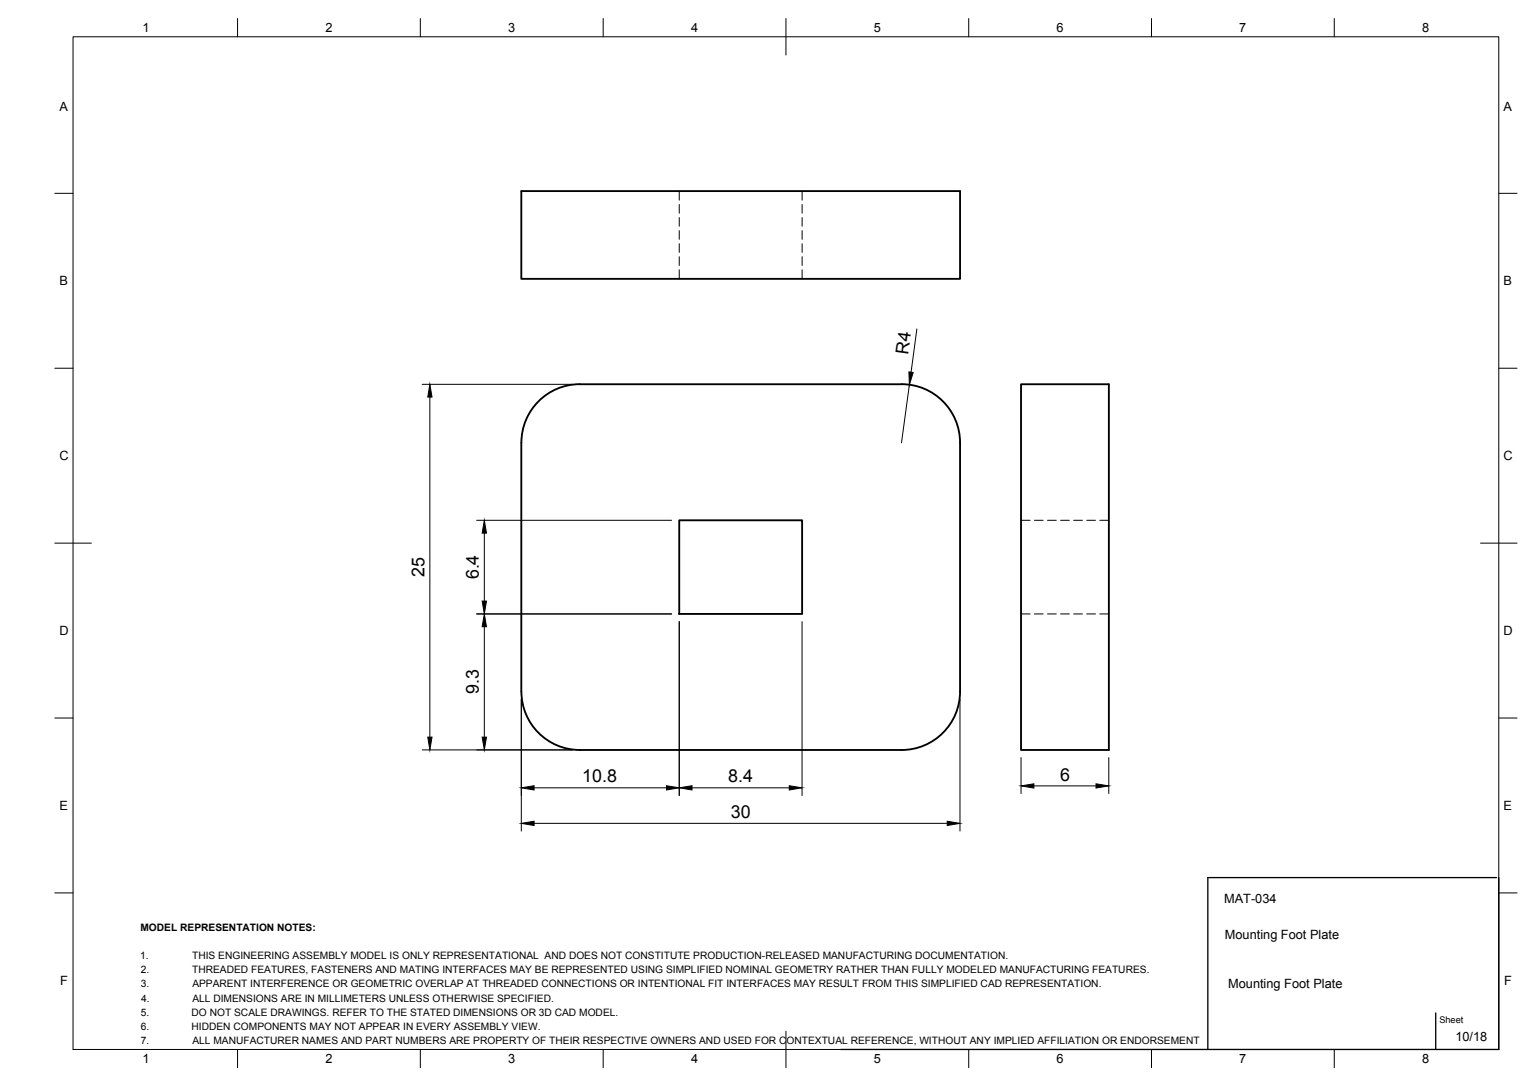
ISO-10303-21;
HEADER;
/* Generated by software containing ST-Developer
 * from STEP Tools, Inc. (www.steptools.com) 
 */

FILE_DESCRIPTION(
/* description */ ('STEP AP214'),
/* implementation_level */ '2;1');

FILE_NAME(
/* name */ 'Mounting Foot Plate.step',
/* time_stamp */ '2026-11-14T09:24:36-08:00',
/* author */ (''),
/* organization */ (''),
/* preprocessor_version */ 'ST-DEVELOPER v20.2',
/* originating_system */ 'Autodesk Translation Framework v15.17.0.0',
/* authorisation */ '');

FILE_SCHEMA (('AUTOMOTIVE_DESIGN { 1 0 10303 214 3 1 1 }'));
ENDSEC;

DATA;
#10=MECHANICAL_DESIGN_GEOMETRIC_PRESENTATION_REPRESENTATION('',(#216),#18867);
#184=SHAPE_REPRESENTATION_RELATIONSHIP('SRR','None',#18948,#200);
#200=ADVANCED_BREP_SHAPE_REPRESENTATION('',(#240),#18864);
#216=STYLED_ITEM('',(#19024),#240);
#240=MANIFOLD_SOLID_BREP('Body1',#10971);
#365=FACE_BOUND('',#1958,.T.);
#366=FACE_BOUND('',#1960,.T.);
#701=PLANE('',#12113);
#702=PLANE('',#12118);
#703=PLANE('',#12123);
#704=PLANE('',#12124);
#705=PLANE('',#12125);
#706=PLANE('',#12126);
#707=PLANE('',#12127);
#708=PLANE('',#12128);
#709=PLANE('',#12129);
#710=PLANE('',#12130);
#1247=FACE_OUTER_BOUND('',#1957,.T.);
#1248=FACE_OUTER_BOUND('',#1959,.T.);
#1249=FACE_OUTER_BOUND('',#1961,.T.);
#1250=FACE_OUTER_BOUND('',#1962,.T.);
#1251=FACE_OUTER_BOUND('',#1963,.T.);
#1252=FACE_OUTER_BOUND('',#1964,.T.);
#1253=FACE_OUTER_BOUND('',#1965,.T.);
#1254=FACE_OUTER_BOUND('',#1966,.T.);
#1255=FACE_OUTER_BOUND('',#1967,.T.);
#1256=FACE_OUTER_BOUND('',#1968,.T.);
#1257=FACE_OUTER_BOUND('',#1969,.T.);
#1258=FACE_OUTER_BOUND('',#1970,.T.);
#1259=FACE_OUTER_BOUND('',#1971,.T.);
#1260=FACE_OUTER_BOUND('',#1972,.T.);
#1957=EDGE_LOOP('',(#9864,#9865,#9866,#9867,#9868,#9869,#9870,#9871));
#1958=EDGE_LOOP('',(#9872,#9873,#9874,#9875));
#1959=EDGE_LOOP('',(#9876,#9877,#9878,#9879,#9880,#9881,#9882,#9883));
#1960=EDGE_LOOP('',(#9884,#9885,#9886,#9887));
#1961=EDGE_LOOP('',(#9888,#9889,#9890,#9891));
#1962=EDGE_LOOP('',(#9892,#9893,#9894,#9895));
#1963=EDGE_LOOP('',(#9896,#9897,#9898,#9899));
#1964=EDGE_LOOP('',(#9900,#9901,#9902,#9903));
#1965=EDGE_LOOP('',(#9904,#9905,#9906,#9907));
#1966=EDGE_LOOP('',(#9908,#9909,#9910,#9911));
#1967=EDGE_LOOP('',(#9912,#9913,#9914,#9915));
#1968=EDGE_LOOP('',(#9916,#9917,#9918,#9919));
#1969=EDGE_LOOP('',(#9920,#9921,#9922,#9923));
#1970=EDGE_LOOP('',(#9924,#9925,#9926,#9927));
#1971=EDGE_LOOP('',(#9928,#9929,#9930,#9931));
#1972=EDGE_LOOP('',(#9932,#9933,#9934,#9935));
#3004=LINE('',#18489,#4018);
#3005=LINE('',#18493,#4019);
#3006=LINE('',#18497,#4020);
#3007=LINE('',#18501,#4021);
#3008=LINE('',#18505,#4022);
#3009=LINE('',#18507,#4023);
#3010=LINE('',#18509,#4024);
#3011=LINE('',#18510,#4025);
#3012=LINE('',#18514,#4026);
#3013=LINE('',#18518,#4027);
#3014=LINE('',#18522,#4028);
#3015=LINE('',#18526,#4029);
#3016=LINE('',#18530,#4030);
#3017=LINE('',#18532,#4031);
#3018=LINE('',#18534,#4032);
#3019=LINE('',#18535,#4033);
#3020=LINE('',#18537,#4034);
#3021=LINE('',#18538,#4035);
#3022=LINE('',#18540,#4036);
#3023=LINE('',#18541,#4037);
#3024=LINE('',#18543,#4038);
#3025=LINE('',#18544,#4039);
#3026=LINE('',#18546,#4040);
#3027=LINE('',#18547,#4041);
#3028=LINE('',#18549,#4042);
#3029=LINE('',#18550,#4043);
#3030=LINE('',#18552,#4044);
#3031=LINE('',#18554,#4045);
#4018=VECTOR('',#15170,1000.);
#4019=VECTOR('',#15173,1000.);
#4020=VECTOR('',#15176,1000.);
#4021=VECTOR('',#15179,1000.);
#4022=VECTOR('',#15182,1000.);
#4023=VECTOR('',#15183,1000.);
#4024=VECTOR('',#15184,1000.);
#4025=VECTOR('',#15185,1000.);
#4026=VECTOR('',#15188,1000.);
#4027=VECTOR('',#15191,1000.);
#4028=VECTOR('',#15194,1000.);
#4029=VECTOR('',#15197,1000.);
#4030=VECTOR('',#15200,1000.);
#4031=VECTOR('',#15201,1000.);
#4032=VECTOR('',#15202,1000.);
#4033=VECTOR('',#15203,1000.);
#4034=VECTOR('',#15206,1000.);
#4035=VECTOR('',#15207,1000.);
#4036=VECTOR('',#15210,1000.);
#4037=VECTOR('',#15211,1000.);
#4038=VECTOR('',#15214,1000.);
#4039=VECTOR('',#15215,1000.);
#4040=VECTOR('',#15218,1000.);
#4041=VECTOR('',#15219,1000.);
#4042=VECTOR('',#15222,1000.);
#4043=VECTOR('',#15223,1000.);
#4044=VECTOR('',#15226,1000.);
#4045=VECTOR('',#15229,1000.);
#4488=CIRCLE('',#12114,4.);
#4489=CIRCLE('',#12115,4.);
#4490=CIRCLE('',#12116,4.);
#4491=CIRCLE('',#12117,4.);
#4492=CIRCLE('',#12119,4.);
#4493=CIRCLE('',#12120,4.);
#4494=CIRCLE('',#12121,4.);
#4495=CIRCLE('',#12122,4.);
#5488=VERTEX_POINT('',#18487);
#5489=VERTEX_POINT('',#18488);
#5490=VERTEX_POINT('',#18490);
#5491=VERTEX_POINT('',#18492);
#5492=VERTEX_POINT('',#18494);
#5493=VERTEX_POINT('',#18496);
#5494=VERTEX_POINT('',#18498);
#5495=VERTEX_POINT('',#18500);
#5496=VERTEX_POINT('',#18503);
#5497=VERTEX_POINT('',#18504);
#5498=VERTEX_POINT('',#18506);
#5499=VERTEX_POINT('',#18508);
#5500=VERTEX_POINT('',#18512);
#5501=VERTEX_POINT('',#18513);
#5502=VERTEX_POINT('',#18515);
#5503=VERTEX_POINT('',#18517);
#5504=VERTEX_POINT('',#18519);
#5505=VERTEX_POINT('',#18521);
#5506=VERTEX_POINT('',#18523);
#5507=VERTEX_POINT('',#18525);
#5508=VERTEX_POINT('',#18528);
#5509=VERTEX_POINT('',#18529);
#5510=VERTEX_POINT('',#18531);
#5511=VERTEX_POINT('',#18533);
#6965=EDGE_CURVE('',#5488,#5489,#3004,.T.);
#6966=EDGE_CURVE('',#5489,#5490,#4488,.T.);
#6967=EDGE_CURVE('',#5490,#5491,#3005,.T.);
#6968=EDGE_CURVE('',#5491,#5492,#4489,.T.);
#6969=EDGE_CURVE('',#5492,#5493,#3006,.T.);
#6970=EDGE_CURVE('',#5493,#5494,#4490,.T.);
#6971=EDGE_CURVE('',#5494,#5495,#3007,.T.);
#6972=EDGE_CURVE('',#5495,#5488,#4491,.T.);
#6973=EDGE_CURVE('',#5496,#5497,#3008,.T.);
#6974=EDGE_CURVE('',#5498,#5496,#3009,.T.);
#6975=EDGE_CURVE('',#5499,#5498,#3010,.T.);
#6976=EDGE_CURVE('',#5497,#5499,#3011,.T.);
#6977=EDGE_CURVE('',#5500,#5501,#3012,.T.);
#6978=EDGE_CURVE('',#5500,#5502,#4492,.T.);
#6979=EDGE_CURVE('',#5503,#5502,#3013,.T.);
#6980=EDGE_CURVE('',#5503,#5504,#4493,.T.);
#6981=EDGE_CURVE('',#5505,#5504,#3014,.T.);
#6982=EDGE_CURVE('',#5505,#5506,#4494,.T.);
#6983=EDGE_CURVE('',#5507,#5506,#3015,.T.);
#6984=EDGE_CURVE('',#5507,#5501,#4495,.T.);
#6985=EDGE_CURVE('',#5508,#5509,#3016,.T.);
#6986=EDGE_CURVE('',#5509,#5510,#3017,.T.);
#6987=EDGE_CURVE('',#5510,#5511,#3018,.T.);
#6988=EDGE_CURVE('',#5511,#5508,#3019,.T.);
#6989=EDGE_CURVE('',#5490,#5500,#3020,.T.);
#6990=EDGE_CURVE('',#5501,#5491,#3021,.T.);
#6991=EDGE_CURVE('',#5492,#5507,#3022,.T.);
#6992=EDGE_CURVE('',#5506,#5493,#3023,.T.);
#6993=EDGE_CURVE('',#5504,#5495,#3024,.T.);
#6994=EDGE_CURVE('',#5494,#5505,#3025,.T.);
#6995=EDGE_CURVE('',#5502,#5489,#3026,.T.);
#6996=EDGE_CURVE('',#5488,#5503,#3027,.T.);
#6997=EDGE_CURVE('',#5498,#5508,#3028,.T.);
#6998=EDGE_CURVE('',#5496,#5509,#3029,.T.);
#6999=EDGE_CURVE('',#5497,#5510,#3030,.T.);
#7000=EDGE_CURVE('',#5499,#5511,#3031,.T.);
#9864=ORIENTED_EDGE('',*,*,#6965,.T.);
#9865=ORIENTED_EDGE('',*,*,#6966,.T.);
#9866=ORIENTED_EDGE('',*,*,#6967,.T.);
#9867=ORIENTED_EDGE('',*,*,#6968,.T.);
#9868=ORIENTED_EDGE('',*,*,#6969,.T.);
#9869=ORIENTED_EDGE('',*,*,#6970,.T.);
#9870=ORIENTED_EDGE('',*,*,#6971,.T.);
#9871=ORIENTED_EDGE('',*,*,#6972,.T.);
#9872=ORIENTED_EDGE('',*,*,#6973,.F.);
#9873=ORIENTED_EDGE('',*,*,#6974,.F.);
#9874=ORIENTED_EDGE('',*,*,#6975,.F.);
#9875=ORIENTED_EDGE('',*,*,#6976,.F.);
#9876=ORIENTED_EDGE('',*,*,#6977,.F.);
#9877=ORIENTED_EDGE('',*,*,#6978,.T.);
#9878=ORIENTED_EDGE('',*,*,#6979,.F.);
#9879=ORIENTED_EDGE('',*,*,#6980,.T.);
#9880=ORIENTED_EDGE('',*,*,#6981,.F.);
#9881=ORIENTED_EDGE('',*,*,#6982,.T.);
#9882=ORIENTED_EDGE('',*,*,#6983,.F.);
#9883=ORIENTED_EDGE('',*,*,#6984,.T.);
#9884=ORIENTED_EDGE('',*,*,#6985,.T.);
#9885=ORIENTED_EDGE('',*,*,#6986,.T.);
#9886=ORIENTED_EDGE('',*,*,#6987,.T.);
#9887=ORIENTED_EDGE('',*,*,#6988,.T.);
#9888=ORIENTED_EDGE('',*,*,#6967,.F.);
#9889=ORIENTED_EDGE('',*,*,#6989,.T.);
#9890=ORIENTED_EDGE('',*,*,#6977,.T.);
#9891=ORIENTED_EDGE('',*,*,#6990,.T.);
#9892=ORIENTED_EDGE('',*,*,#6969,.F.);
#9893=ORIENTED_EDGE('',*,*,#6991,.T.);
#9894=ORIENTED_EDGE('',*,*,#6983,.T.);
#9895=ORIENTED_EDGE('',*,*,#6992,.T.);
#9896=ORIENTED_EDGE('',*,*,#6981,.T.);
#9897=ORIENTED_EDGE('',*,*,#6993,.T.);
#9898=ORIENTED_EDGE('',*,*,#6971,.F.);
#9899=ORIENTED_EDGE('',*,*,#6994,.T.);
#9900=ORIENTED_EDGE('',*,*,#6979,.T.);
#9901=ORIENTED_EDGE('',*,*,#6995,.T.);
#9902=ORIENTED_EDGE('',*,*,#6965,.F.);
#9903=ORIENTED_EDGE('',*,*,#6996,.T.);
#9904=ORIENTED_EDGE('',*,*,#6985,.F.);
#9905=ORIENTED_EDGE('',*,*,#6997,.F.);
#9906=ORIENTED_EDGE('',*,*,#6974,.T.);
#9907=ORIENTED_EDGE('',*,*,#6998,.T.);
#9908=ORIENTED_EDGE('',*,*,#6986,.F.);
#9909=ORIENTED_EDGE('',*,*,#6998,.F.);
#9910=ORIENTED_EDGE('',*,*,#6973,.T.);
#9911=ORIENTED_EDGE('',*,*,#6999,.T.);
#9912=ORIENTED_EDGE('',*,*,#6987,.F.);
#9913=ORIENTED_EDGE('',*,*,#6999,.F.);
#9914=ORIENTED_EDGE('',*,*,#6976,.T.);
#9915=ORIENTED_EDGE('',*,*,#7000,.T.);
#9916=ORIENTED_EDGE('',*,*,#6988,.F.);
#9917=ORIENTED_EDGE('',*,*,#7000,.F.);
#9918=ORIENTED_EDGE('',*,*,#6975,.T.);
#9919=ORIENTED_EDGE('',*,*,#6997,.T.);
#9920=ORIENTED_EDGE('',*,*,#6966,.F.);
#9921=ORIENTED_EDGE('',*,*,#6995,.F.);
#9922=ORIENTED_EDGE('',*,*,#6978,.F.);
#9923=ORIENTED_EDGE('',*,*,#6989,.F.);
#9924=ORIENTED_EDGE('',*,*,#6972,.F.);
#9925=ORIENTED_EDGE('',*,*,#6993,.F.);
#9926=ORIENTED_EDGE('',*,*,#6980,.F.);
#9927=ORIENTED_EDGE('',*,*,#6996,.F.);
#9928=ORIENTED_EDGE('',*,*,#6968,.F.);
#9929=ORIENTED_EDGE('',*,*,#6990,.F.);
#9930=ORIENTED_EDGE('',*,*,#6984,.F.);
#9931=ORIENTED_EDGE('',*,*,#6991,.F.);
#9932=ORIENTED_EDGE('',*,*,#6970,.F.);
#9933=ORIENTED_EDGE('',*,*,#6992,.F.);
#9934=ORIENTED_EDGE('',*,*,#6982,.F.);
#9935=ORIENTED_EDGE('',*,*,#6994,.F.);
#10341=CYLINDRICAL_SURFACE('',#12131,4.);
#10342=CYLINDRICAL_SURFACE('',#12132,4.);
#10343=CYLINDRICAL_SURFACE('',#12133,4.);
#10344=CYLINDRICAL_SURFACE('',#12134,4.);
#10884=ADVANCED_FACE('',(#1247,#365),#701,.T.);
#10885=ADVANCED_FACE('',(#1248,#366),#702,.F.);
#10886=ADVANCED_FACE('',(#1249),#703,.F.);
#10887=ADVANCED_FACE('',(#1250),#704,.F.);
#10888=ADVANCED_FACE('',(#1251),#705,.F.);
#10889=ADVANCED_FACE('',(#1252),#706,.F.);
#10890=ADVANCED_FACE('',(#1253),#707,.T.);
#10891=ADVANCED_FACE('',(#1254),#708,.T.);
#10892=ADVANCED_FACE('',(#1255),#709,.T.);
#10893=ADVANCED_FACE('',(#1256),#710,.T.);
#10894=ADVANCED_FACE('',(#1257),#10341,.T.);
#10895=ADVANCED_FACE('',(#1258),#10342,.T.);
#10896=ADVANCED_FACE('',(#1259),#10343,.T.);
#10897=ADVANCED_FACE('',(#1260),#10344,.T.);
#10971=CLOSED_SHELL('',(#10884,#10885,#10886,#10887,#10888,#10889,#10890,
#10891,#10892,#10893,#10894,#10895,#10896,#10897));
#12112=AXIS2_PLACEMENT_3D('',#18485,#15166,#15167);
#12113=AXIS2_PLACEMENT_3D('',#18486,#15168,#15169);
#12114=AXIS2_PLACEMENT_3D('',#18491,#15171,#15172);
#12115=AXIS2_PLACEMENT_3D('',#18495,#15174,#15175);
#12116=AXIS2_PLACEMENT_3D('',#18499,#15177,#15178);
#12117=AXIS2_PLACEMENT_3D('',#18502,#15180,#15181);
#12118=AXIS2_PLACEMENT_3D('',#18511,#15186,#15187);
#12119=AXIS2_PLACEMENT_3D('',#18516,#15189,#15190);
#12120=AXIS2_PLACEMENT_3D('',#18520,#15192,#15193);
#12121=AXIS2_PLACEMENT_3D('',#18524,#15195,#15196);
#12122=AXIS2_PLACEMENT_3D('',#18527,#15198,#15199);
#12123=AXIS2_PLACEMENT_3D('',#18536,#15204,#15205);
#12124=AXIS2_PLACEMENT_3D('',#18539,#15208,#15209);
#12125=AXIS2_PLACEMENT_3D('',#18542,#15212,#15213);
#12126=AXIS2_PLACEMENT_3D('',#18545,#15216,#15217);
#12127=AXIS2_PLACEMENT_3D('',#18548,#15220,#15221);
#12128=AXIS2_PLACEMENT_3D('',#18551,#15224,#15225);
#12129=AXIS2_PLACEMENT_3D('',#18553,#15227,#15228);
#12130=AXIS2_PLACEMENT_3D('',#18555,#15230,#15231);
#12131=AXIS2_PLACEMENT_3D('',#18556,#15232,#15233);
#12132=AXIS2_PLACEMENT_3D('',#18557,#15234,#15235);
#12133=AXIS2_PLACEMENT_3D('',#18558,#15236,#15237);
#12134=AXIS2_PLACEMENT_3D('',#18559,#15238,#15239);
#15166=DIRECTION('axis',(0.,0.,1.));
#15167=DIRECTION('refdir',(1.,0.,0.));
#15168=DIRECTION('center_axis',(0.,1.,0.));
#15169=DIRECTION('ref_axis',(0.,0.,1.));
#15170=DIRECTION('',(-1.,0.,1.15648231731787E-16));
#15171=DIRECTION('center_axis',(0.,1.,0.));
#15172=DIRECTION('ref_axis',(0.,0.,1.));
#15173=DIRECTION('',(0.,0.,1.));
#15174=DIRECTION('center_axis',(0.,1.,0.));
#15175=DIRECTION('ref_axis',(0.,0.,1.));
#15176=DIRECTION('',(1.,0.,-1.15648231731787E-16));
#15177=DIRECTION('center_axis',(0.,1.,0.));
#15178=DIRECTION('ref_axis',(0.,0.,1.));
#15179=DIRECTION('',(0.,0.,-1.));
#15180=DIRECTION('center_axis',(0.,1.,0.));
#15181=DIRECTION('ref_axis',(0.,0.,1.));
#15182=DIRECTION('',(1.,0.,-1.03257349760524E-16));
#15183=DIRECTION('',(0.,0.,1.));
#15184=DIRECTION('',(-1.,0.,1.03257349760524E-16));
#15185=DIRECTION('',(0.,0.,-1.));
#15186=DIRECTION('center_axis',(0.,1.,0.));
#15187=DIRECTION('ref_axis',(0.,0.,1.));
#15188=DIRECTION('',(0.,0.,1.));
#15189=DIRECTION('center_axis',(0.,-1.,0.));
#15190=DIRECTION('ref_axis',(0.,0.,1.));
#15191=DIRECTION('',(-1.,0.,1.15648231731787E-16));
#15192=DIRECTION('center_axis',(0.,-1.,0.));
#15193=DIRECTION('ref_axis',(0.,0.,1.));
#15194=DIRECTION('',(0.,0.,-1.));
#15195=DIRECTION('center_axis',(0.,-1.,0.));
#15196=DIRECTION('ref_axis',(0.,0.,1.));
#15197=DIRECTION('',(1.,0.,-1.15648231731787E-16));
#15198=DIRECTION('center_axis',(0.,-1.,0.));
#15199=DIRECTION('ref_axis',(0.,0.,1.));
#15200=DIRECTION('',(0.,0.,1.));
#15201=DIRECTION('',(1.,0.,-1.03257349760524E-16));
#15202=DIRECTION('',(0.,0.,-1.));
#15203=DIRECTION('',(-1.,0.,1.03257349760524E-16));
#15204=DIRECTION('center_axis',(1.,0.,0.));
#15205=DIRECTION('ref_axis',(0.,0.,-1.));
#15206=DIRECTION('',(0.,-1.,0.));
#15207=DIRECTION('',(0.,1.,0.));
#15208=DIRECTION('center_axis',(-1.15648231731787E-16,0.,-1.));
#15209=DIRECTION('ref_axis',(-1.,0.,1.15648231731787E-16));
#15210=DIRECTION('',(0.,-1.,0.));
#15211=DIRECTION('',(0.,1.,0.));
#15212=DIRECTION('center_axis',(-1.,0.,0.));
#15213=DIRECTION('ref_axis',(0.,0.,1.));
#15214=DIRECTION('',(0.,1.,0.));
#15215=DIRECTION('',(0.,-1.,0.));
#15216=DIRECTION('center_axis',(1.15648231731787E-16,0.,1.));
#15217=DIRECTION('ref_axis',(1.,0.,-1.15648231731787E-16));
#15218=DIRECTION('',(0.,1.,0.));
#15219=DIRECTION('',(0.,-1.,0.));
#15220=DIRECTION('center_axis',(1.,0.,0.));
#15221=DIRECTION('ref_axis',(0.,0.,-1.));
#15222=DIRECTION('',(0.,-1.,0.));
#15223=DIRECTION('',(0.,-1.,0.));
#15224=DIRECTION('center_axis',(-1.03257349760524E-16,0.,-1.));
#15225=DIRECTION('ref_axis',(-1.,0.,1.03257349760524E-16));
#15226=DIRECTION('',(0.,-1.,0.));
#15227=DIRECTION('center_axis',(-1.,0.,0.));
#15228=DIRECTION('ref_axis',(0.,0.,1.));
#15229=DIRECTION('',(0.,-1.,0.));
#15230=DIRECTION('center_axis',(1.03257349760524E-16,0.,1.));
#15231=DIRECTION('ref_axis',(1.,0.,-1.03257349760524E-16));
#15232=DIRECTION('center_axis',(0.,-1.,0.));
#15233=DIRECTION('ref_axis',(0.,0.,-1.));
#15234=DIRECTION('center_axis',(0.,-1.,0.));
#15235=DIRECTION('ref_axis',(0.,0.,-1.));
#15236=DIRECTION('center_axis',(0.,-1.,0.));
#15237=DIRECTION('ref_axis',(0.,0.,-1.));
#15238=DIRECTION('center_axis',(0.,-1.,0.));
#15239=DIRECTION('ref_axis',(0.,0.,-1.));
#18485=CARTESIAN_POINT('',(0.,0.,0.));
#18486=CARTESIAN_POINT('Origin',(0.,6.,0.));
#18487=CARTESIAN_POINT('',(11.,6.,-12.5));
#18488=CARTESIAN_POINT('',(-11.,6.,-12.5));
#18489=CARTESIAN_POINT('',(15.,6.,-12.5));
#18490=CARTESIAN_POINT('',(-15.,6.,-8.49999999999999));
#18491=CARTESIAN_POINT('Origin',(-11.,6.,-8.49999999999999));
#18492=CARTESIAN_POINT('',(-15.,6.,8.50000000000001));
#18493=CARTESIAN_POINT('',(-15.,6.,12.5));
#18494=CARTESIAN_POINT('',(-11.,6.,12.5));
#18495=CARTESIAN_POINT('Origin',(-11.,6.,8.50000000000001));
#18496=CARTESIAN_POINT('',(11.,6.,12.5));
#18497=CARTESIAN_POINT('',(15.,6.,12.5));
#18498=CARTESIAN_POINT('',(15.,6.,8.5));
#18499=CARTESIAN_POINT('Origin',(11.,6.,8.5));
#18500=CARTESIAN_POINT('',(15.,6.,-8.5));
#18501=CARTESIAN_POINT('',(15.,6.,12.5));
#18502=CARTESIAN_POINT('Origin',(11.,6.,-8.5));
#18503=CARTESIAN_POINT('',(-4.2,6.,3.2));
#18504=CARTESIAN_POINT('',(4.2,6.,3.2));
#18505=CARTESIAN_POINT('',(4.2,6.,3.2));
#18506=CARTESIAN_POINT('',(-4.2,6.,-3.2));
#18507=CARTESIAN_POINT('',(-4.2,6.,3.2));
#18508=CARTESIAN_POINT('',(4.2,6.,-3.2));
#18509=CARTESIAN_POINT('',(4.2,6.,-3.2));
#18510=CARTESIAN_POINT('',(4.2,6.,3.2));
#18511=CARTESIAN_POINT('Origin',(0.,0.,0.));
#18512=CARTESIAN_POINT('',(-15.,0.,-8.49999999999999));
#18513=CARTESIAN_POINT('',(-15.,0.,8.50000000000001));
#18514=CARTESIAN_POINT('',(-15.,0.,12.5));
#18515=CARTESIAN_POINT('',(-11.,0.,-12.5));
#18516=CARTESIAN_POINT('Origin',(-11.,0.,-8.49999999999999));
#18517=CARTESIAN_POINT('',(11.,0.,-12.5));
#18518=CARTESIAN_POINT('',(15.,0.,-12.5));
#18519=CARTESIAN_POINT('',(15.,0.,-8.5));
#18520=CARTESIAN_POINT('Origin',(11.,0.,-8.5));
#18521=CARTESIAN_POINT('',(15.,0.,8.5));
#18522=CARTESIAN_POINT('',(15.,0.,12.5));
#18523=CARTESIAN_POINT('',(11.,0.,12.5));
#18524=CARTESIAN_POINT('Origin',(11.,0.,8.5));
#18525=CARTESIAN_POINT('',(-11.,0.,12.5));
#18526=CARTESIAN_POINT('',(15.,0.,12.5));
#18527=CARTESIAN_POINT('Origin',(-11.,0.,8.50000000000001));
#18528=CARTESIAN_POINT('',(-4.2,0.,-3.2));
#18529=CARTESIAN_POINT('',(-4.2,0.,3.2));
#18530=CARTESIAN_POINT('',(-4.2,0.,3.2));
#18531=CARTESIAN_POINT('',(4.2,0.,3.2));
#18532=CARTESIAN_POINT('',(4.2,0.,3.2));
#18533=CARTESIAN_POINT('',(4.2,0.,-3.2));
#18534=CARTESIAN_POINT('',(4.2,0.,3.2));
#18535=CARTESIAN_POINT('',(4.2,0.,-3.2));
#18536=CARTESIAN_POINT('Origin',(-15.,6.,12.5));
#18537=CARTESIAN_POINT('',(-15.,6.,-8.49999999999999));
#18538=CARTESIAN_POINT('',(-15.,6.,8.50000000000001));
#18539=CARTESIAN_POINT('Origin',(15.,6.,12.5));
#18540=CARTESIAN_POINT('',(-11.,6.,12.5));
#18541=CARTESIAN_POINT('',(11.,6.,12.5));
#18542=CARTESIAN_POINT('Origin',(15.,6.,12.5));
#18543=CARTESIAN_POINT('',(15.,6.,-8.5));
#18544=CARTESIAN_POINT('',(15.,6.,8.5));
#18545=CARTESIAN_POINT('Origin',(15.,6.,-12.5));
#18546=CARTESIAN_POINT('',(-11.,6.,-12.5));
#18547=CARTESIAN_POINT('',(11.,6.,-12.5));
#18548=CARTESIAN_POINT('Origin',(-4.2,6.,3.2));
#18549=CARTESIAN_POINT('',(-4.2,6.,-3.2));
#18550=CARTESIAN_POINT('',(-4.2,6.,3.2));
#18551=CARTESIAN_POINT('Origin',(4.2,6.,3.2));
#18552=CARTESIAN_POINT('',(4.2,6.,3.2));
#18553=CARTESIAN_POINT('Origin',(4.2,6.,3.2));
#18554=CARTESIAN_POINT('',(4.2,6.,-3.2));
#18555=CARTESIAN_POINT('Origin',(4.2,6.,-3.2));
#18556=CARTESIAN_POINT('Origin',(-11.,6.,-8.49999999999999));
#18557=CARTESIAN_POINT('Origin',(11.,6.,-8.5));
#18558=CARTESIAN_POINT('Origin',(-11.,6.,8.50000000000001));
#18559=CARTESIAN_POINT('Origin',(11.,6.,8.5));
#18846=UNCERTAINTY_MEASURE_WITH_UNIT(LENGTH_MEASURE(0.01),#18868,
'DISTANCE_ACCURACY_VALUE',
'Maximum model space distance between geometric entities at asserted c
onnectivities');
#18849=UNCERTAINTY_MEASURE_WITH_UNIT(LENGTH_MEASURE(0.01),#18868,
'DISTANCE_ACCURACY_VALUE',
'Maximum model space distance between geometric entities at asserted c
onnectivities');
#18864=(
GEOMETRIC_REPRESENTATION_CONTEXT(3)
GLOBAL_UNCERTAINTY_ASSIGNED_CONTEXT((#18846))
GLOBAL_UNIT_ASSIGNED_CONTEXT((#18868,#18870,#18871))
REPRESENTATION_CONTEXT('','3D')
);
#18867=(
GEOMETRIC_REPRESENTATION_CONTEXT(3)
GLOBAL_UNCERTAINTY_ASSIGNED_CONTEXT((#18849))
GLOBAL_UNIT_ASSIGNED_CONTEXT((#18868,#18870,#18871))
REPRESENTATION_CONTEXT('','3D')
);
#18868=(
LENGTH_UNIT()
NAMED_UNIT(*)
SI_UNIT(.MILLI.,.METRE.)
);
#18870=(
NAMED_UNIT(*)
PLANE_ANGLE_UNIT()
SI_UNIT($,.RADIAN.)
);
#18871=(
NAMED_UNIT(*)
SI_UNIT($,.STERADIAN.)
SOLID_ANGLE_UNIT()
);
#18886=SHAPE_DEFINITION_REPRESENTATION(#18903,#18948);
#18903=PRODUCT_DEFINITION_SHAPE('',$,#18966);
#18948=SHAPE_REPRESENTATION('',(#12112),#18864);
#18951=PRODUCT_DEFINITION_CONTEXT('part definition',#19004,'design');
#18966=PRODUCT_DEFINITION('Mounting Foot Plate','Mounting Foot Plate',#18983,
#18951);
#18983=PRODUCT_DEFINITION_FORMATION('',$,#19020);
#19004=APPLICATION_CONTEXT(
'Core Data for Automotive Mechanical Design Process');
#19005=PRODUCT_CONTEXT('part definition',#19004,'mechanical');
#19020=PRODUCT('Mounting Foot Plate','Mounting Foot Plate',$,(#19005));
#19024=PRESENTATION_STYLE_ASSIGNMENT((#19030));
#19030=SURFACE_STYLE_USAGE(.BOTH.,#19036);
#19036=SURFACE_SIDE_STYLE('',(#19042));
#19042=SURFACE_STYLE_FILL_AREA(#19048);
#19048=FILL_AREA_STYLE('Opaque(20,51,87)',(#19054));
#19054=FILL_AREA_STYLE_COLOUR('Opaque(20,51,87)',#19060);
#19060=COLOUR_RGB('Opaque(20,51,87)',0.0784313725490196,0.2,0.341176470588235);
ENDSEC;
END-ISO-10303-21;
